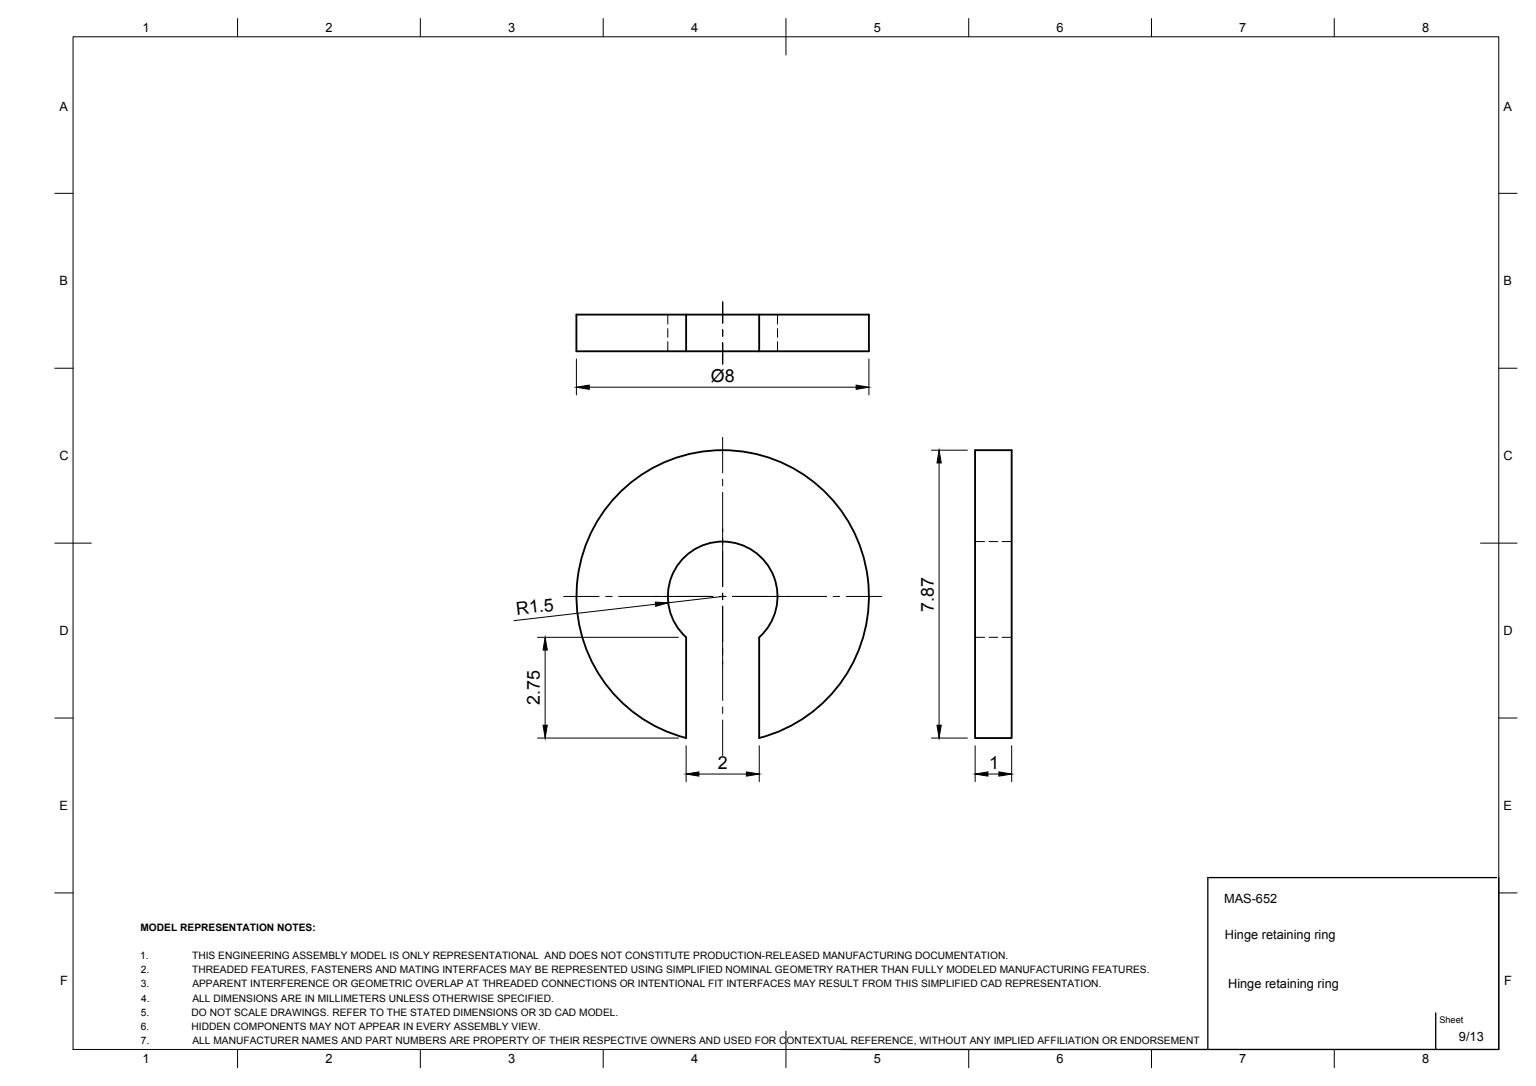
ISO-10303-21;
HEADER;
/* Generated by software containing ST-Developer
 * from STEP Tools, Inc. (www.steptools.com) 
 */

FILE_DESCRIPTION(
/* description */ ('Independent hinged machine back cover with retained hinge pins, perim
eter gasket and quarter-turn cam latch. Nominal cover 360 x 260 x 3 mm
, frame 430 x 300 x 20 mm. No guarding, structural or ingress rating a
ssigned.'),
/* implementation_level */ '2;1');

FILE_NAME(
/* name */ 'Hinge retaining ring.step',
/* time_stamp */ '2026-11-09T19:36:59-08:00',
/* author */ (''),
/* organization */ (''),
/* preprocessor_version */ 'ST-DEVELOPER v20.2',
/* originating_system */ 'Autodesk Translation Framework v15.17.0.0',
/* authorisation */ '');

FILE_SCHEMA (('AUTOMOTIVE_DESIGN { 1 0 10303 214 3 1 1 }'));
ENDSEC;

DATA;
#10=MECHANICAL_DESIGN_GEOMETRIC_PRESENTATION_REPRESENTATION('',(#209),#32627);
#173=SHAPE_REPRESENTATION_RELATIONSHIP('SRR','None',#32719,#191);
#191=ADVANCED_BREP_SHAPE_REPRESENTATION('',(#227),#32620);
#209=STYLED_ITEM('',(#32809),#227);
#227=MANIFOLD_SOLID_BREP('Body1',#8686);
#407=PLANE('',#9313);
#408=PLANE('',#9314);
#409=PLANE('',#9315);
#410=PLANE('',#9322);
#786=FACE_OUTER_BOUND('',#1304,.T.);
#787=FACE_OUTER_BOUND('',#1305,.T.);
#788=FACE_OUTER_BOUND('',#1306,.T.);
#789=FACE_OUTER_BOUND('',#1307,.T.);
#790=FACE_OUTER_BOUND('',#1308,.T.);
#791=FACE_OUTER_BOUND('',#1309,.T.);
#1304=EDGE_LOOP('',(#7149,#7150,#7151,#7152));
#1305=EDGE_LOOP('',(#7153,#7154,#7155,#7156));
#1306=EDGE_LOOP('',(#7157,#7158,#7159,#7160));
#1307=EDGE_LOOP('',(#7161,#7162,#7163,#7164));
#1308=EDGE_LOOP('',(#7165,#7166,#7167,#7168));
#1309=EDGE_LOOP('',(#7169,#7170,#7171,#7172));
#1547=CIRCLE('',#9316,4.);
#1548=CIRCLE('',#9317,1.5);
#1549=CIRCLE('',#9319,1.5);
#1550=CIRCLE('',#9321,4.);
#2556=LINE('',#26289,#3102);
#2557=LINE('',#26291,#3103);
#2558=LINE('',#26293,#3104);
#2559=LINE('',#26294,#3105);
#2560=LINE('',#26298,#3106);
#2561=LINE('',#26300,#3107);
#2562=LINE('',#26302,#3108);
#2563=LINE('',#26303,#3109);
#3102=VECTOR('',#10754,10.);
#3103=VECTOR('',#10755,10.);
#3104=VECTOR('',#10756,10.);
#3105=VECTOR('',#10757,10.);
#3106=VECTOR('',#10760,10.);
#3107=VECTOR('',#10761,10.);
#3108=VECTOR('',#10762,10.);
#3109=VECTOR('',#10763,10.);
#3861=VERTEX_POINT('',#26287);
#3862=VERTEX_POINT('',#26288);
#3863=VERTEX_POINT('',#26290);
#3864=VERTEX_POINT('',#26292);
#3865=VERTEX_POINT('',#26296);
#3866=VERTEX_POINT('',#26297);
#3867=VERTEX_POINT('',#26299);
#3868=VERTEX_POINT('',#26301);
#4998=EDGE_CURVE('',#3861,#3862,#2556,.T.);
#4999=EDGE_CURVE('',#3863,#3861,#2557,.T.);
#5000=EDGE_CURVE('',#3864,#3863,#2558,.T.);
#5001=EDGE_CURVE('',#3862,#3864,#2559,.T.);
#5002=EDGE_CURVE('',#3865,#3866,#2560,.T.);
#5003=EDGE_CURVE('',#3867,#3865,#2561,.T.);
#5004=EDGE_CURVE('',#3868,#3867,#2562,.T.);
#5005=EDGE_CURVE('',#3866,#3868,#2563,.T.);
#5006=EDGE_CURVE('',#3863,#3868,#1547,.T.);
#5007=EDGE_CURVE('',#3866,#3861,#1548,.T.);
#5008=EDGE_CURVE('',#3865,#3862,#1549,.T.);
#5009=EDGE_CURVE('',#3864,#3867,#1550,.T.);
#7149=ORIENTED_EDGE('',*,*,#4998,.F.);
#7150=ORIENTED_EDGE('',*,*,#4999,.F.);
#7151=ORIENTED_EDGE('',*,*,#5000,.F.);
#7152=ORIENTED_EDGE('',*,*,#5001,.F.);
#7153=ORIENTED_EDGE('',*,*,#5002,.F.);
#7154=ORIENTED_EDGE('',*,*,#5003,.F.);
#7155=ORIENTED_EDGE('',*,*,#5004,.F.);
#7156=ORIENTED_EDGE('',*,*,#5005,.F.);
#7157=ORIENTED_EDGE('',*,*,#5005,.T.);
#7158=ORIENTED_EDGE('',*,*,#5006,.F.);
#7159=ORIENTED_EDGE('',*,*,#4999,.T.);
#7160=ORIENTED_EDGE('',*,*,#5007,.F.);
#7161=ORIENTED_EDGE('',*,*,#5002,.T.);
#7162=ORIENTED_EDGE('',*,*,#5007,.T.);
#7163=ORIENTED_EDGE('',*,*,#4998,.T.);
#7164=ORIENTED_EDGE('',*,*,#5008,.F.);
#7165=ORIENTED_EDGE('',*,*,#5004,.T.);
#7166=ORIENTED_EDGE('',*,*,#5009,.F.);
#7167=ORIENTED_EDGE('',*,*,#5000,.T.);
#7168=ORIENTED_EDGE('',*,*,#5006,.T.);
#7169=ORIENTED_EDGE('',*,*,#5003,.T.);
#7170=ORIENTED_EDGE('',*,*,#5008,.T.);
#7171=ORIENTED_EDGE('',*,*,#5001,.T.);
#7172=ORIENTED_EDGE('',*,*,#5009,.T.);
#8112=CYLINDRICAL_SURFACE('',#9318,1.5);
#8113=CYLINDRICAL_SURFACE('',#9320,4.);
#8534=ADVANCED_FACE('',(#786),#407,.F.);
#8535=ADVANCED_FACE('',(#787),#408,.F.);
#8536=ADVANCED_FACE('',(#788),#409,.F.);
#8537=ADVANCED_FACE('',(#789),#8112,.F.);
#8538=ADVANCED_FACE('',(#790),#8113,.T.);
#8539=ADVANCED_FACE('',(#791),#410,.T.);
#8686=CLOSED_SHELL('',(#8534,#8535,#8536,#8537,#8538,#8539));
#9312=AXIS2_PLACEMENT_3D('',#26285,#10750,#10751);
#9313=AXIS2_PLACEMENT_3D('',#26286,#10752,#10753);
#9314=AXIS2_PLACEMENT_3D('',#26295,#10758,#10759);
#9315=AXIS2_PLACEMENT_3D('',#26304,#10764,#10765);
#9316=AXIS2_PLACEMENT_3D('',#26305,#10766,#10767);
#9317=AXIS2_PLACEMENT_3D('',#26306,#10768,#10769);
#9318=AXIS2_PLACEMENT_3D('',#26307,#10770,#10771);
#9319=AXIS2_PLACEMENT_3D('',#26308,#10772,#10773);
#9320=AXIS2_PLACEMENT_3D('',#26309,#10774,#10775);
#9321=AXIS2_PLACEMENT_3D('',#26310,#10776,#10777);
#9322=AXIS2_PLACEMENT_3D('',#26311,#10778,#10779);
#10750=DIRECTION('axis',(0.,0.,1.));
#10751=DIRECTION('refdir',(1.,0.,0.));
#10752=DIRECTION('center_axis',(-1.,0.,0.));
#10753=DIRECTION('ref_axis',(0.,1.,0.));
#10754=DIRECTION('',(0.,0.,1.));
#10755=DIRECTION('',(0.,-1.,0.));
#10756=DIRECTION('',(0.,0.,-1.));
#10757=DIRECTION('',(0.,1.,0.));
#10758=DIRECTION('center_axis',(1.,0.,0.));
#10759=DIRECTION('ref_axis',(0.,-1.,0.));
#10760=DIRECTION('',(0.,0.,-1.));
#10761=DIRECTION('',(0.,-1.,0.));
#10762=DIRECTION('',(0.,0.,1.));
#10763=DIRECTION('',(0.,1.,0.));
#10764=DIRECTION('center_axis',(0.,0.,1.));
#10765=DIRECTION('ref_axis',(1.,0.,0.));
#10766=DIRECTION('center_axis',(0.,0.,1.));
#10767=DIRECTION('ref_axis',(1.,0.,0.));
#10768=DIRECTION('center_axis',(0.,0.,-1.));
#10769=DIRECTION('ref_axis',(1.,0.,0.));
#10770=DIRECTION('center_axis',(0.,0.,1.));
#10771=DIRECTION('ref_axis',(6.12323399573677E-17,-1.,0.));
#10772=DIRECTION('center_axis',(0.,0.,-1.));
#10773=DIRECTION('ref_axis',(1.,0.,0.));
#10774=DIRECTION('center_axis',(0.,0.,1.));
#10775=DIRECTION('ref_axis',(6.12323399573677E-17,-1.,0.));
#10776=DIRECTION('center_axis',(0.,0.,1.));
#10777=DIRECTION('ref_axis',(1.,0.,0.));
#10778=DIRECTION('center_axis',(0.,0.,1.));
#10779=DIRECTION('ref_axis',(1.,0.,0.));
#26285=CARTESIAN_POINT('',(0.,0.,0.));
#26286=CARTESIAN_POINT('Origin',(-1.,0.,1.));
#26287=CARTESIAN_POINT('',(-1.,1.11803398874989,0.));
#26288=CARTESIAN_POINT('',(-1.,1.11803398874989,1.));
#26289=CARTESIAN_POINT('',(-1.,1.11803398874989,0.));
#26290=CARTESIAN_POINT('',(-1.,3.87298334620742,0.));
#26291=CARTESIAN_POINT('',(-1.,0.,0.));
#26292=CARTESIAN_POINT('',(-1.,3.87298334620742,1.));
#26293=CARTESIAN_POINT('',(-1.,3.87298334620742,0.));
#26294=CARTESIAN_POINT('',(-1.,0.,1.));
#26295=CARTESIAN_POINT('Origin',(1.,8.,1.));
#26296=CARTESIAN_POINT('',(1.,1.11803398874989,1.));
#26297=CARTESIAN_POINT('',(1.,1.11803398874989,0.));
#26298=CARTESIAN_POINT('',(1.,1.11803398874989,0.));
#26299=CARTESIAN_POINT('',(1.,3.87298334620742,1.));
#26300=CARTESIAN_POINT('',(1.,4.,1.));
#26301=CARTESIAN_POINT('',(1.,3.87298334620742,0.));
#26302=CARTESIAN_POINT('',(1.,3.87298334620742,0.));
#26303=CARTESIAN_POINT('',(1.,4.,0.));
#26304=CARTESIAN_POINT('Origin',(0.,0.,0.));
#26305=CARTESIAN_POINT('Origin',(0.,0.,0.));
#26306=CARTESIAN_POINT('Origin',(0.,0.,0.));
#26307=CARTESIAN_POINT('Origin',(0.,0.,0.));
#26308=CARTESIAN_POINT('Origin',(0.,0.,1.));
#26309=CARTESIAN_POINT('Origin',(0.,0.,0.));
#26310=CARTESIAN_POINT('Origin',(0.,0.,1.));
#26311=CARTESIAN_POINT('Origin',(0.,0.,1.));
#32600=UNCERTAINTY_MEASURE_WITH_UNIT(LENGTH_MEASURE(0.01),#32628,
'DISTANCE_ACCURACY_VALUE',
'Maximum model space distance between geometric entities at asserted c
onnectivities');
#32607=UNCERTAINTY_MEASURE_WITH_UNIT(LENGTH_MEASURE(0.01),#32628,
'DISTANCE_ACCURACY_VALUE',
'Maximum model space distance between geometric entities at asserted c
onnectivities');
#32620=(
GEOMETRIC_REPRESENTATION_CONTEXT(3)
GLOBAL_UNCERTAINTY_ASSIGNED_CONTEXT((#32600))
GLOBAL_UNIT_ASSIGNED_CONTEXT((#32628,#32630,#32631))
REPRESENTATION_CONTEXT('','3D')
);
#32627=(
GEOMETRIC_REPRESENTATION_CONTEXT(3)
GLOBAL_UNCERTAINTY_ASSIGNED_CONTEXT((#32607))
GLOBAL_UNIT_ASSIGNED_CONTEXT((#32628,#32630,#32631))
REPRESENTATION_CONTEXT('','3D')
);
#32628=(
LENGTH_UNIT()
NAMED_UNIT(*)
SI_UNIT(.MILLI.,.METRE.)
);
#32630=(
NAMED_UNIT(*)
PLANE_ANGLE_UNIT()
SI_UNIT($,.RADIAN.)
);
#32631=(
NAMED_UNIT(*)
SI_UNIT($,.STERADIAN.)
SOLID_ANGLE_UNIT()
);
#32644=SHAPE_DEFINITION_REPRESENTATION(#32663,#32719);
#32663=PRODUCT_DEFINITION_SHAPE('',$,#32739);
#32719=SHAPE_REPRESENTATION('',(#9312),#32620);
#32726=PRODUCT_DEFINITION_CONTEXT('part definition',#32785,'design');
#32739=PRODUCT_DEFINITION('Hinge retaining ring','Hinge retaining ring',
#32758,#32726);
#32758=PRODUCT_DEFINITION_FORMATION('',$,#32799);
#32785=APPLICATION_CONTEXT(
'Core Data for Automotive Mechanical Design Process');
#32786=PRODUCT_CONTEXT('part definition',#32785,'mechanical');
#32799=PRODUCT('Hinge retaining ring','Hinge retaining ring',$,(#32786));
#32809=PRESENTATION_STYLE_ASSIGNMENT((#32816));
#32816=SURFACE_STYLE_USAGE(.BOTH.,#32823);
#32823=SURFACE_SIDE_STYLE('',(#32830));
#32830=SURFACE_STYLE_FILL_AREA(#32837);
#32837=FILL_AREA_STYLE('Dark gray',(#32844));
#32844=FILL_AREA_STYLE_COLOUR('Dark gray',#32851);
#32851=COLOUR_RGB('Dark gray',0.250980392156863,0.282352941176471,0.32156862745098);
ENDSEC;
END-ISO-10303-21;
